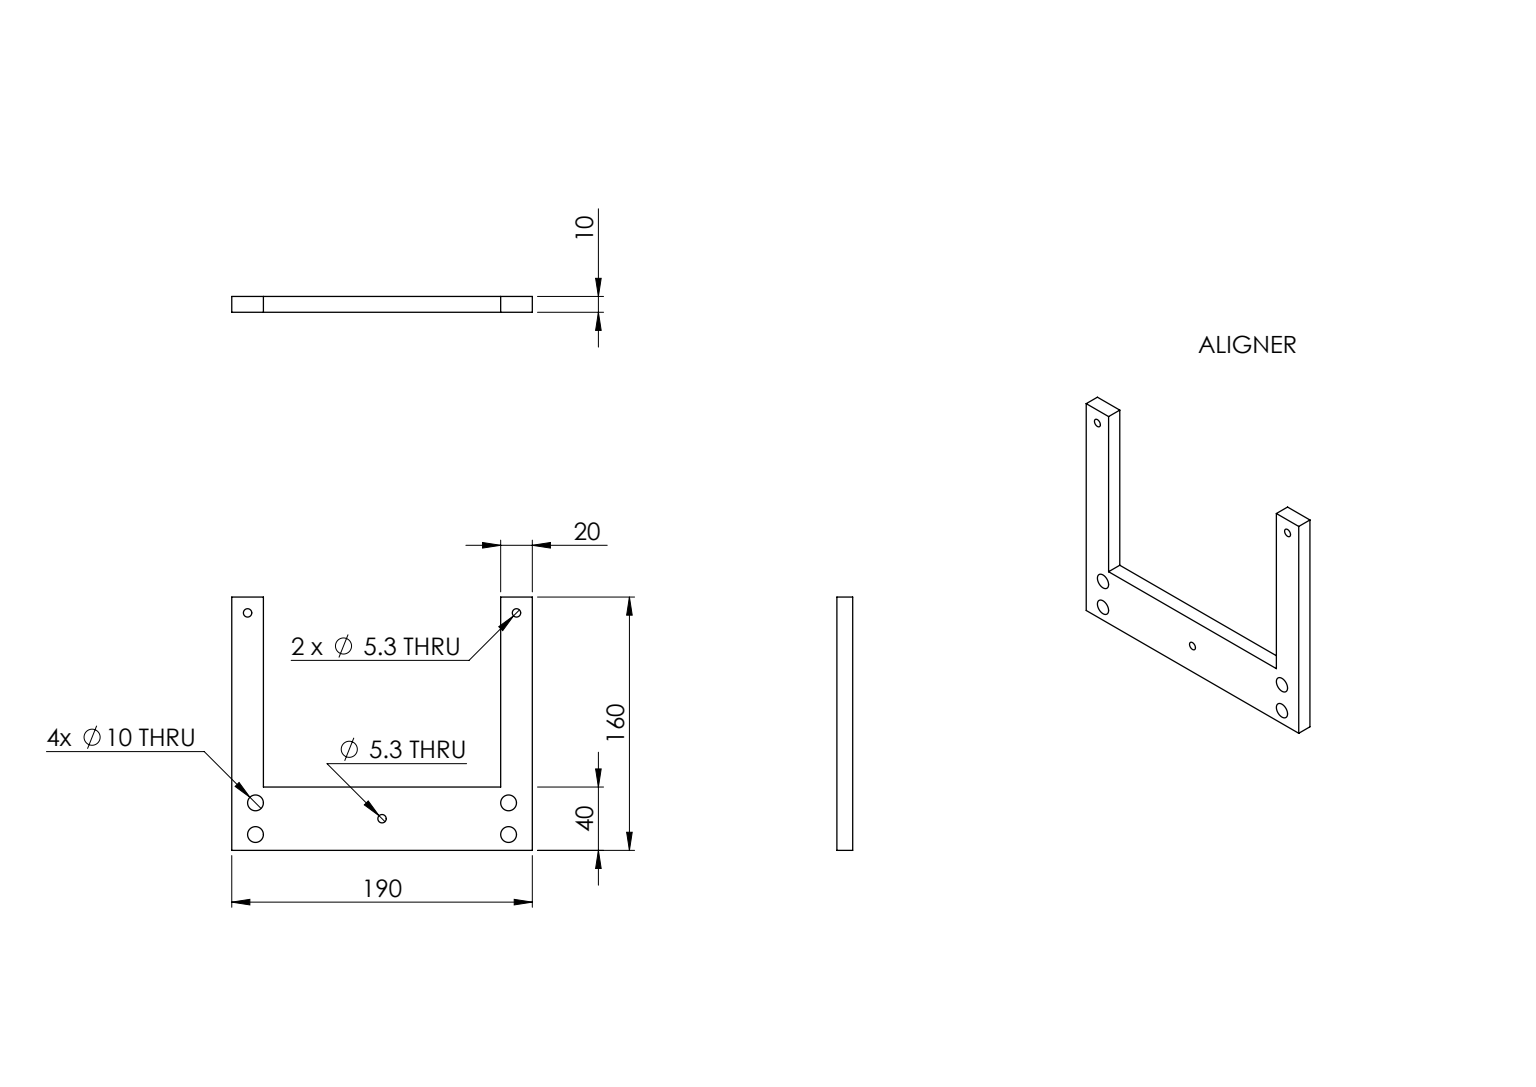
ISO-10303-21;
HEADER;
FILE_DESCRIPTION (('STEP AP214'),
    '1' );
FILE_NAME ('aligner.step',
    '2026-10-24T13:33:06',
    ( '' ),
    ( '' ),
    'SwSTEP 2.0',
    'SolidWorks 2026',
    '' );
FILE_SCHEMA (( 'AUTOMOTIVE_DESIGN' ));
ENDSEC;

DATA;
#23=ORIENTED_EDGE ( 'NONE', *, *, #5278, .F. ) ;
#39=ORIENTED_EDGE ( 'NONE', *, *, #7804, .T. ) ;
#91=ADVANCED_FACE ( 'NONE', ( #1003 ), #2259, .T. ) ;
#92=CARTESIAN_POINT ( 'NONE',  ( -144.9999999999999432, -105.0000000000000853, 40.00000000000000000 ) ) ;
#103=DIRECTION ( 'NONE',  ( -1.000000000000000000, 0.000000000000000000, 0.000000000000000000 ) ) ;
#109=SURFACE_STYLE_FILL_AREA ( #5656 ) ;
#110=EDGE_CURVE ( 'NONE', #13194, #10462, #10760, .T. ) ;
#136=EDGE_LOOP ( 'NONE', ( #496, #11440, #13448, #1824 ) ) ;
#153=PLANE ( 'NONE',  #6564 ) ;
#202=DIRECTION ( 'NONE',  ( -0.000000000000000000, 0.000000000000000000, -1.000000000000000000 ) ) ;
#219=CIRCLE ( 'NONE', #5381, 5.000000000000004441 ) ;
#220=AXIS2_PLACEMENT_3D ( 'NONE', #2707, #9091, #281 ) ;
#224=CARTESIAN_POINT ( 'NONE',  ( -219.9999999999999147, -85.00000000000009948, 30.00000000000000000 ) ) ;
#238=EDGE_CURVE ( 'NONE', #5881, #9436, #12617, .T. ) ;
#248=DIRECTION ( 'NONE',  ( -0.000000000000000000, -0.000000000000000000, -1.000000000000000000 ) ) ;
#250=DIRECTION ( 'NONE',  ( 1.000000000000000000, 0.000000000000000000, 0.000000000000000000 ) ) ;
#251=EDGE_CURVE ( 'NONE', #12108, #865, #13488, .T. ) ;
#281=DIRECTION ( 'NONE',  ( 0.000000000000000000, 0.000000000000000000, -1.000000000000000000 ) ) ;
#287=DIRECTION ( 'NONE',  ( -0.000000000000000000, -1.000000000000000000, -0.000000000000000000 ) ) ;
#291=PRODUCT_DEFINITION_SHAPE ( 'NONE', 'NONE',  #3819 ) ;
#312=CARTESIAN_POINT ( 'NONE',  ( -304.9999999999999432, 45.00000000000001421, 30.00000000000000000 ) ) ;
#323=EDGE_LOOP ( 'NONE', ( #13718, #1656 ) ) ;
#332=FACE_OUTER_BOUND ( 'NONE', #8846, .T. ) ;
#341=CIRCLE ( 'NONE', #14262, 2.649999999999985700 ) ;
#353=FACE_BOUND ( 'NONE', #877, .T. ) ;
#354=AXIS2_PLACEMENT_3D ( 'NONE', #6912, #4747, #11272 ) ;
#367=LINE ( 'NONE', #8152, #5578 ) ;
#369=MECHANICAL_DESIGN_GEOMETRIC_PRESENTATION_REPRESENTATION('',(#7806),#10136);
#403=ORIENTED_EDGE ( 'NONE', *, *, #10858, .T. ) ;
#413=ADVANCED_FACE ( 'NONE', ( #5943 ), #5008, .F. ) ;
#417=VERTEX_POINT ( 'NONE', #3915 ) ;
#420=ORIENTED_EDGE ( 'NONE', *, *, #110, .F. ) ;
#422=ORIENTED_EDGE ( 'NONE', *, *, #251, .T. ) ;
#432=AXIS2_PLACEMENT_3D ( 'NONE', #6019, #1877, #3778 ) ;
#438=ORIENTED_EDGE ( 'NONE', *, *, #6313, .F. ) ;
#442=DIRECTION ( 'NONE',  ( -1.000000000000000000, 0.000000000000000000, 0.000000000000000000 ) ) ;
#450=ADVANCED_FACE ( 'NONE', ( #1804 ), #8183, .F. ) ;
#473=AXIS2_PLACEMENT_3D ( 'NONE', #9647, #5162, #2982 ) ;
#475=DIRECTION ( 'NONE',  ( -1.000000000000000000, 0.000000000000000000, 0.000000000000000000 ) ) ;
#477=EDGE_LOOP ( 'NONE', ( #11769, #9508 ) ) ;
#479=CARTESIAN_POINT ( 'NONE',  ( -299.9999999999999432, -95.00000000000008527, 354.1421356237308942 ) ) ;
#496=ORIENTED_EDGE ( 'NONE', *, *, #11704, .F. ) ;
#499=DIRECTION ( 'NONE',  ( 0.000000000000000000, 0.000000000000000000, -1.000000000000000000 ) ) ;
#508=FACE_OUTER_BOUND ( 'NONE', #3187, .T. ) ;
#520=CARTESIAN_POINT ( 'NONE',  ( -144.9999999999999432, -105.0000000000000853, 40.00000000000000000 ) ) ;
#528=ADVANCED_FACE ( 'NONE', ( #2680 ), #11531, .F. ) ;
#543=LINE ( 'NONE', #10288, #10586 ) ;
#547=DIRECTION ( 'NONE',  ( 0.000000000000000000, -0.000000000000000000, 1.000000000000000000 ) ) ;
#555=ORIENTED_EDGE ( 'NONE', *, *, #6914, .F. ) ;
#575=DIRECTION ( 'NONE',  ( 1.000000000000000000, 7.304098846218135653E-17, -0.000000000000000000 ) ) ;
#592=PLANE ( 'NONE',  #11528 ) ;
#598=AXIS2_PLACEMENT_3D ( 'NONE', #11123, #1157, #11993 ) ;
#606=ORIENTED_EDGE ( 'NONE', *, *, #1377, .T. ) ;
#608=AXIS2_PLACEMENT_3D ( 'NONE', #4664, #202, #3506 ) ;
#609=LINE ( 'NONE', #2598, #1621 ) ;
#652=ORIENTED_EDGE ( 'NONE', *, *, #7099, .T. ) ;
#663=VERTEX_POINT ( 'NONE', #2017 ) ;
#740=CARTESIAN_POINT ( 'NONE',  ( -304.9999999999999432, -75.00000000000008527, 39.99999999999997868 ) ) ;
#741=CYLINDRICAL_SURFACE ( 'NONE', #5392, 2.649999999999985700 ) ;
#775=DIRECTION ( 'NONE',  ( -1.000000000000000000, 0.000000000000000000, 0.000000000000000000 ) ) ;
#777=ORIENTED_EDGE ( 'NONE', *, *, #7329, .T. ) ;
#820=EDGE_LOOP ( 'NONE', ( #4312, #1747, #10761, #1441 ) ) ;
#852=( LENGTH_UNIT ( ) NAMED_UNIT ( * ) SI_UNIT ( .MILLI., .METRE. ) );
#863=EDGE_LOOP ( 'NONE', ( #12473, #1825 ) ) ;
#865=VERTEX_POINT ( 'NONE', #13683 ) ;
#877=EDGE_LOOP ( 'NONE', ( #5483, #13862 ) ) ;
#904=ORIENTED_EDGE ( 'NONE', *, *, #1524, .T. ) ;
#971=AXIS2_PLACEMENT_3D ( 'NONE', #12444, #13808, #8300 ) ;
#981=VERTEX_POINT ( 'NONE', #9708 ) ;
#998=DIRECTION ( 'NONE',  ( 1.000000000000000000, 0.000000000000000000, 0.000000000000000000 ) ) ;
#1003=FACE_OUTER_BOUND ( 'NONE', #2000, .T. ) ;
#1034=CIRCLE ( 'NONE', #14250, 5.000000000000004441 ) ;
#1087=DIRECTION ( 'NONE',  ( 0.000000000000000000, 1.000000000000000000, 0.000000000000000000 ) ) ;
#1090=CARTESIAN_POINT ( 'NONE',  ( -140.0000000000000000, -95.00000000000008527, 40.00000000000000000 ) ) ;
#1122=VECTOR ( 'NONE', #11092, 1000.000000000000000 ) ;
#1157=DIRECTION ( 'NONE',  ( -0.000000000000000000, -0.000000000000000000, -1.000000000000000000 ) ) ;
#1160=CYLINDRICAL_SURFACE ( 'NONE', #8697, 5.000000000000004441 ) ;
#1167=CARTESIAN_POINT ( 'NONE',  ( -314.9999999999999432, 55.00000000000001421, 30.00000000000000000 ) ) ;
#1174=ADVANCED_FACE ( 'NONE', ( #7983 ), #4410, .T. ) ;
#1191=VECTOR ( 'NONE', #7717, 1000.000000000000000 ) ;
#1214=DIRECTION ( 'NONE',  ( 0.000000000000000000, -0.000000000000000000, 1.000000000000000000 ) ) ;
#1247=CARTESIAN_POINT ( 'NONE',  ( -124.9999999999999432, -105.0000000000000853, 40.00000000000000000 ) ) ;
#1276=ORIENTED_EDGE ( 'NONE', *, *, #9037, .T. ) ;
#1299=EDGE_CURVE ( 'NONE', #13972, #8006, #4015, .T. ) ;
#1300=CIRCLE ( 'NONE', #6183, 5.000000000000004441 ) ;
#1347=PRODUCT ( 'aligner', 'aligner', '', ( #6175 ) ) ;
#1353=CARTESIAN_POINT ( 'NONE',  ( -314.9999999999999432, -105.0000000000000995, 40.00000000000000000 ) ) ;
#1354=DIRECTION ( 'NONE',  ( -0.000000000000000000, -0.000000000000000000, -1.000000000000000000 ) ) ;
#1377=EDGE_CURVE ( 'NONE', #5028, #10577, #8861, .T. ) ;
#1406=CARTESIAN_POINT ( 'NONE',  ( -294.9999999999999432, -75.00000000000008527, 39.99999999999997868 ) ) ;
#1414=DIRECTION ( 'NONE',  ( -0.000000000000000000, -0.000000000000000000, -1.000000000000000000 ) ) ;
#1441=ORIENTED_EDGE ( 'NONE', *, *, #12534, .T. ) ;
#1459=ORIENTED_EDGE ( 'NONE', *, *, #6313, .T. ) ;
#1512=EDGE_CURVE ( 'NONE', #4493, #865, #13215, .T. ) ;
#1524=EDGE_CURVE ( 'NONE', #6598, #3716, #12128, .T. ) ;
#1530=AXIS2_PLACEMENT_3D ( 'NONE', #9386, #12937, #7060 ) ;
#1569=CARTESIAN_POINT ( 'NONE',  ( -140.0000000000000000, -75.00000000000008527, 30.00000000000000000 ) ) ;
#1582=ORIENTED_EDGE ( 'NONE', *, *, #8645, .T. ) ;
#1621=VECTOR ( 'NONE', #6943, 1000.000000000000000 ) ;
#1631=CARTESIAN_POINT ( 'NONE',  ( -134.9999999999999716, 45.00000000000001421, 30.00000000000000000 ) ) ;
#1649=CIRCLE ( 'NONE', #473, 5.000000000000004441 ) ;
#1653=ORIENTED_EDGE ( 'NONE', *, *, #8448, .T. ) ;
#1655=CYLINDRICAL_SURFACE ( 'NONE', #5562, 5.000000000000004441 ) ;
#1656=ORIENTED_EDGE ( 'NONE', *, *, #12195, .T. ) ;
#1691=CARTESIAN_POINT ( 'NONE',  ( -294.9999999999999432, -75.00000000000008527, 354.1421356237308942 ) ) ;
#1695=EDGE_CURVE ( 'NONE', #7212, #9436, #2619, .T. ) ;
#1718=DIRECTION ( 'NONE',  ( -0.000000000000000000, 0.000000000000000000, -1.000000000000000000 ) ) ;
#1723=CARTESIAN_POINT ( 'NONE',  ( -299.9999999999999432, -75.00000000000008527, 354.1421356237308942 ) ) ;
#1725=DIRECTION ( 'NONE',  ( -0.000000000000000000, -0.000000000000000000, -1.000000000000000000 ) ) ;
#1745=ORIENTED_EDGE ( 'NONE', *, *, #4492, .F. ) ;
#1747=ORIENTED_EDGE ( 'NONE', *, *, #5401, .T. ) ;
#1766=CARTESIAN_POINT ( 'NONE',  ( -294.9999999999999432, -65.00000000000011369, 30.00000000000000000 ) ) ;
#1773=FACE_BOUND ( 'NONE', #3437, .T. ) ;
#1781=ORIENTED_EDGE ( 'NONE', *, *, #1695, .T. ) ;
#1804=FACE_OUTER_BOUND ( 'NONE', #8996, .T. ) ;
#1810=VERTEX_POINT ( 'NONE', #2905 ) ;
#1824=ORIENTED_EDGE ( 'NONE', *, *, #4456, .T. ) ;
#1825=ORIENTED_EDGE ( 'NONE', *, *, #5920, .F. ) ;
#1875=ORIENTED_EDGE ( 'NONE', *, *, #7549, .T. ) ;
#1877=DIRECTION ( 'NONE',  ( -0.000000000000000000, 0.000000000000000000, -1.000000000000000000 ) ) ;
#1878=EDGE_CURVE ( 'NONE', #13081, #11113, #4181, .T. ) ;
#1879=ADVANCED_FACE ( 'NONE', ( #10446 ), #1655, .F. ) ;
#1887=CARTESIAN_POINT ( 'NONE',  ( -219.9999999999999147, -85.00000000000009948, 30.00000000000000000 ) ) ;
#1965=CARTESIAN_POINT ( 'NONE',  ( -124.9999999999999432, 55.00000000000001421, 40.00000000000000000 ) ) ;
#1973=DIRECTION ( 'NONE',  ( -1.000000000000000000, -7.304098846218135653E-17, 0.000000000000000000 ) ) ;
#1975=DIRECTION ( 'NONE',  ( -0.000000000000000000, 0.000000000000000000, -1.000000000000000000 ) ) ;
#1978=AXIS2_PLACEMENT_3D ( 'NONE', #6016, #10442, #475 ) ;
#1982=VERTEX_POINT ( 'NONE', #12040 ) ;
#1987=FACE_OUTER_BOUND ( 'NONE', #13855, .T. ) ;
#1993=FACE_BOUND ( 'NONE', #863, .T. ) ;
#2000=EDGE_LOOP ( 'NONE', ( #1745, #12037, #3225, #9323 ) ) ;
#2004=VECTOR ( 'NONE', #287, 1000.000000000000000 ) ;
#2017=CARTESIAN_POINT ( 'NONE',  ( -307.6499999999999204, 45.00000000000001421, 40.00000000000000000 ) ) ;
#2064=CARTESIAN_POINT ( 'NONE',  ( -294.9999999999999432, -65.00000000000011369, 40.00000000000000000 ) ) ;
#2072=DIRECTION ( 'NONE',  ( -1.000000000000000000, 0.000000000000000000, 0.000000000000000000 ) ) ;
#2098=EDGE_LOOP ( 'NONE', ( #8207, #7792 ) ) ;
#2112=ORIENTED_EDGE ( 'NONE', *, *, #1524, .F. ) ;
#2125=CIRCLE ( 'NONE', #3735, 2.649999999999985700 ) ;
#2137=ORIENTED_EDGE ( 'NONE', *, *, #7283, .T. ) ;
#2148=LINE ( 'NONE', #2289, #6717 ) ;
#2186=DIRECTION ( 'NONE',  ( -1.000000000000000000, -1.460819769243627131E-16, 0.000000000000000000 ) ) ;
#2211=DIRECTION ( 'NONE',  ( -1.000000000000000000, 0.000000000000000000, 0.000000000000000000 ) ) ;
#2239=VERTEX_POINT ( 'NONE', #7655 ) ;
#2248=AXIS2_PLACEMENT_3D ( 'NONE', #13499, #6762, #4521 ) ;
#2259=PLANE ( 'NONE',  #4981 ) ;
#2262=CIRCLE ( 'NONE', #7126, 2.649999999999985700 ) ;
#2265=ORIENTED_EDGE ( 'NONE', *, *, #5401, .F. ) ;
#2271=DIRECTION ( 'NONE',  ( -0.000000000000000000, 0.000000000000000000, -1.000000000000000000 ) ) ;
#2289=CARTESIAN_POINT ( 'NONE',  ( -132.3499999999999943, 45.00000000000001421, 30.00000000000000000 ) ) ;
#2322=FILL_AREA_STYLE_COLOUR ( '', #10495 ) ;
#2336=VERTEX_POINT ( 'NONE', #4687 ) ;
#2355=DIRECTION ( 'NONE',  ( 1.000000000000000000, 0.000000000000000000, 0.000000000000000000 ) ) ;
#2382=PRODUCT_DEFINITION_FORMATION_WITH_SPECIFIED_SOURCE ( 'ANY', '', #1347, .NOT_KNOWN. ) ;
#2383=ORIENTED_EDGE ( 'NONE', *, *, #12018, .T. ) ;
#2389=VECTOR ( 'NONE', #11604, 1000.000000000000000 ) ;
#2401=ORIENTED_EDGE ( 'NONE', *, *, #6755, .F. ) ;
#2408=CARTESIAN_POINT ( 'NONE',  ( -144.9999999999999432, -105.0000000000000853, 30.00000000000000000 ) ) ;
#2415=ORIENTED_EDGE ( 'NONE', *, *, #10083, .F. ) ;
#2468=ORIENTED_EDGE ( 'NONE', *, *, #13310, .F. ) ;
#2505=LINE ( 'NONE', #6918, #8854 ) ;
#2507=LINE ( 'NONE', #3524, #6486 ) ;
#2513=EDGE_CURVE ( 'NONE', #13072, #981, #4528, .T. ) ;
#2533=VECTOR ( 'NONE', #11742, 1000.000000000000000 ) ;
#2540=VERTEX_POINT ( 'NONE', #12002 ) ;
#2577=DIRECTION ( 'NONE',  ( -0.000000000000000000, -0.000000000000000000, -1.000000000000000000 ) ) ;
#2598=CARTESIAN_POINT ( 'NONE',  ( -124.9999999999999432, -65.00000000000008527, 30.00000000000000000 ) ) ;
#2609=DIRECTION ( 'NONE',  ( 1.000000000000000000, 0.000000000000000000, 0.000000000000000000 ) ) ;
#2613=EDGE_LOOP ( 'NONE', ( #438, #8269, #2615, #12189 ) ) ;
#2615=ORIENTED_EDGE ( 'NONE', *, *, #10294, .T. ) ;
#2619=LINE ( 'NONE', #10158, #7237 ) ;
#2679=ORIENTED_EDGE ( 'NONE', *, *, #12960, .F. ) ;
#2680=FACE_OUTER_BOUND ( 'NONE', #6752, .T. ) ;
#2707=CARTESIAN_POINT ( 'NONE',  ( -294.9999999999999432, -105.0000000000000853, 40.00000000000000000 ) ) ;
#2779=ORIENTED_EDGE ( 'NONE', *, *, #6667, .T. ) ;
#2787=PLANE ( 'NONE',  #9424 ) ;
#2801=ORIENTED_EDGE ( 'NONE', *, *, #4387, .T. ) ;
#2833=VECTOR ( 'NONE', #3291, 1000.000000000000000 ) ;
#2853=ORIENTED_EDGE ( 'NONE', *, *, #2513, .F. ) ;
#2887=VERTEX_POINT ( 'NONE', #5103 ) ;
#2895=LINE ( 'NONE', #9572, #2533 ) ;
#2905=CARTESIAN_POINT ( 'NONE',  ( -222.6499999999998920, -85.00000000000009948, 30.00000000000000000 ) ) ;
#2909=EDGE_LOOP ( 'NONE', ( #12132, #1459, #6840, #3447 ) ) ;
#2927=FACE_OUTER_BOUND ( 'NONE', #11134, .T. ) ;
#2930=FACE_BOUND ( 'NONE', #10179, .T. ) ;
#2942=CIRCLE ( 'NONE', #3179, 5.000000000000004441 ) ;
#2949=CARTESIAN_POINT ( 'NONE',  ( -144.9999999999999432, -65.00000000000008527, 40.00000000000000000 ) ) ;
#2982=DIRECTION ( 'NONE',  ( 1.000000000000000000, 0.000000000000000000, 0.000000000000000000 ) ) ;
#3019=ORIENTED_EDGE ( 'NONE', *, *, #1299, .T. ) ;
#3021=CARTESIAN_POINT ( 'NONE',  ( -314.9999999999999432, -105.0000000000000995, 40.00000000000000000 ) ) ;
#3028=FACE_BOUND ( 'NONE', #9601, .T. ) ;
#3040=ORIENTED_EDGE ( 'NONE', *, *, #11028, .F. ) ;
#3062=CARTESIAN_POINT ( 'NONE',  ( -132.3499999999999943, 45.00000000000001421, 30.00000000000000000 ) ) ;
#3106=FACE_BOUND ( 'NONE', #12537, .T. ) ;
#3120=DIRECTION ( 'NONE',  ( 1.000000000000000000, 0.000000000000000000, 0.000000000000000000 ) ) ;
#3123=ORIENTED_EDGE ( 'NONE', *, *, #6292, .T. ) ;
#3179=AXIS2_PLACEMENT_3D ( 'NONE', #8521, #6352, #10782 ) ;
#3187=EDGE_LOOP ( 'NONE', ( #1582, #6980, #3939, #6808 ) ) ;
#3211=VECTOR ( 'NONE', #9099, 1000.000000000000000 ) ;
#3225=ORIENTED_EDGE ( 'NONE', *, *, #10052, .T. ) ;
#3246=VECTOR ( 'NONE', #13387, 1000.000000000000000 ) ;
#3291=DIRECTION ( 'NONE',  ( 1.000000000000000000, 7.304098846218135653E-17, -0.000000000000000000 ) ) ;
#3321=CARTESIAN_POINT ( 'NONE',  ( -304.9999999999999432, 45.00000000000001421, 30.00000000000000000 ) ) ;
#3339=EDGE_CURVE ( 'NONE', #2239, #5230, #5127, .T. ) ;
#3369=DIRECTION ( 'NONE',  ( -0.000000000000000000, 0.000000000000000000, -1.000000000000000000 ) ) ;
#3373=DIRECTION ( 'NONE',  ( 1.000000000000000000, 0.000000000000000000, 0.000000000000000000 ) ) ;
#3437=EDGE_LOOP ( 'NONE', ( #13630, #12058 ) ) ;
#3447=ORIENTED_EDGE ( 'NONE', *, *, #10294, .F. ) ;
#3457=CIRCLE ( 'NONE', #6920, 5.000000000000004441 ) ;
#3464=DIRECTION ( 'NONE',  ( 0.000000000000000000, 1.000000000000000000, 0.000000000000000000 ) ) ;
#3506=DIRECTION ( 'NONE',  ( 1.000000000000000000, 0.000000000000000000, 0.000000000000000000 ) ) ;
#3524=CARTESIAN_POINT ( 'NONE',  ( -307.6499999999999204, 45.00000000000001421, 30.00000000000000000 ) ) ;
#3560=CARTESIAN_POINT ( 'NONE',  ( -124.9999999999999432, -105.0000000000000853, 40.00000000000000000 ) ) ;
#3627=CIRCLE ( 'NONE', #8729, 5.000000000000004441 ) ;
#3639=CIRCLE ( 'NONE', #598, 2.649999999999985700 ) ;
#3708=DIRECTION ( 'NONE',  ( -0.000000000000000000, -0.000000000000000000, -1.000000000000000000 ) ) ;
#3716=VERTEX_POINT ( 'NONE', #1167 ) ;
#3724=FACE_BOUND ( 'NONE', #323, .T. ) ;
#3727=LINE ( 'NONE', #9923, #2004 ) ;
#3731=CARTESIAN_POINT ( 'NONE',  ( -307.6499999999999204, 45.00000000000001421, 30.00000000000000000 ) ) ;
#3735=AXIS2_PLACEMENT_3D ( 'NONE', #5207, #9622, #2072 ) ;
#3764=CARTESIAN_POINT ( 'NONE',  ( -124.9999999999999432, 55.00000000000001421, 30.00000000000000000 ) ) ;
#3778=DIRECTION ( 'NONE',  ( 1.000000000000000000, 0.000000000000000000, 0.000000000000000000 ) ) ;
#3799=LINE ( 'NONE', #9315, #10831 ) ;
#3809=DIRECTION ( 'NONE',  ( -0.000000000000000000, -0.000000000000000000, -1.000000000000000000 ) ) ;
#3810=CLOSED_SHELL ( 'NONE', ( #7980, #528, #10284, #12528, #450, #11788, #1879, #11864, #12453, #9342, #5261, #6691, #9234, #1174, #4628, #13130, #91, #6937, #10572, #13117, #413, #6012, #13880, #14110 ) ) ;
#3818=CYLINDRICAL_SURFACE ( 'NONE', #10112, 2.649999999999985700 ) ;
#3819=PRODUCT_DEFINITION ( 'UNKNOWN', '', #2382, #6290 ) ;
#3864=CIRCLE ( 'NONE', #11976, 2.649999999999985700 ) ;
#3877=LINE ( 'NONE', #4090, #7803 ) ;
#3915=CARTESIAN_POINT ( 'NONE',  ( -217.3499999999999375, -85.00000000000009948, 30.00000000000000000 ) ) ;
#3939=ORIENTED_EDGE ( 'NONE', *, *, #5202, .T. ) ;
#3953=DIRECTION ( 'NONE',  ( -0.000000000000000000, -0.000000000000000000, -1.000000000000000000 ) ) ;
#3963=FACE_BOUND ( 'NONE', #14205, .T. ) ;
#3986=EDGE_CURVE ( 'NONE', #6598, #13972, #13276, .T. ) ;
#4015=LINE ( 'NONE', #7129, #10195 ) ;
#4057=DIRECTION ( 'NONE',  ( 1.000000000000000000, 0.000000000000000000, 0.000000000000000000 ) ) ;
#4065=DIRECTION ( 'NONE',  ( 0.000000000000000000, -0.000000000000000000, 1.000000000000000000 ) ) ;
#4085=AXIS2_PLACEMENT_3D ( 'NONE', #6459, #4065, #11759 ) ;
#4090=CARTESIAN_POINT ( 'NONE',  ( -217.3499999999999375, -85.00000000000009948, 30.00000000000000000 ) ) ;
#4102=DIRECTION ( 'NONE',  ( -0.000000000000000000, -0.000000000000000000, -1.000000000000000000 ) ) ;
#4124=ORIENTED_EDGE ( 'NONE', *, *, #3339, .F. ) ;
#4136=DIRECTION ( 'NONE',  ( -0.000000000000000000, 0.000000000000000000, -1.000000000000000000 ) ) ;
#4181=CIRCLE ( 'NONE', #432, 5.000000000000004441 ) ;
#4188=VECTOR ( 'NONE', #12173, 1000.000000000000000 ) ;
#4218=LINE ( 'NONE', #12050, #11760 ) ;
#4228=DIRECTION ( 'NONE',  ( 0.000000000000000000, -0.000000000000000000, 1.000000000000000000 ) ) ;
#4256=VERTEX_POINT ( 'NONE', #8178 ) ;
#4257=FACE_BOUND ( 'NONE', #9141, .T. ) ;
#4290=DIRECTION ( 'NONE',  ( 0.000000000000000000, 0.000000000000000000, -1.000000000000000000 ) ) ;
#4295=CARTESIAN_POINT ( 'NONE',  ( -140.0000000000000000, -75.00000000000008527, 40.00000000000000000 ) ) ;
#4312=ORIENTED_EDGE ( 'NONE', *, *, #5068, .F. ) ;
#4343=CIRCLE ( 'NONE', #10844, 2.649999999999985700 ) ;
#4359=UNCERTAINTY_MEASURE_WITH_UNIT (LENGTH_MEASURE( 1.000000000000000082E-05 ), #7754, 'distance_accuracy_value', 'NONE');
#4379=DIRECTION ( 'NONE',  ( -1.000000000000000000, 0.000000000000000000, 0.000000000000000000 ) ) ;
#4387=EDGE_CURVE ( 'NONE', #7915, #7212, #3457, .T. ) ;
#4410=PLANE ( 'NONE',  #220 ) ;
#4437=( NAMED_UNIT ( * ) SI_UNIT ( $, .STERADIAN. ) SOLID_ANGLE_UNIT ( ) );
#4451=LINE ( 'NONE', #2408, #11517 ) ;
#4456=EDGE_CURVE ( 'NONE', #13972, #10462, #2895, .T. ) ;
#4459=ORIENTED_EDGE ( 'NONE', *, *, #10381, .T. ) ;
#4479=( GEOMETRIC_REPRESENTATION_CONTEXT ( 3 ) GLOBAL_UNCERTAINTY_ASSIGNED_CONTEXT ( ( #9868 ) ) GLOBAL_UNIT_ASSIGNED_CONTEXT ( ( #5519, #4648, #4437 ) ) REPRESENTATION_CONTEXT ( 'NONE', 'WORKASPACE' ) );
#4492=EDGE_CURVE ( 'NONE', #12063, #9564, #13320, .T. ) ;
#4493=VERTEX_POINT ( 'NONE', #7801 ) ;
#4521=DIRECTION ( 'NONE',  ( 1.000000000000000000, 0.000000000000000000, 0.000000000000000000 ) ) ;
#4528=CIRCLE ( 'NONE', #12618, 5.000000000000004441 ) ;
#4535=EDGE_CURVE ( 'NONE', #11936, #11113, #8762, .T. ) ;
#4586=FACE_OUTER_BOUND ( 'NONE', #14222, .T. ) ;
#4606=DIRECTION ( 'NONE',  ( 0.000000000000000000, 0.000000000000000000, 1.000000000000000000 ) ) ;
#4620=LINE ( 'NONE', #10197, #8516 ) ;
#4623=PLANE ( 'NONE',  #6927 ) ;
#4628=ADVANCED_FACE ( 'NONE', ( #8088 ), #4623, .T. ) ;
#4648=( NAMED_UNIT ( * ) PLANE_ANGLE_UNIT ( ) SI_UNIT ( $, .RADIAN. ) );
#4664=CARTESIAN_POINT ( 'NONE',  ( -140.0000000000000000, -95.00000000000008527, 30.00000000000000000 ) ) ;
#4675=LINE ( 'NONE', #8331, #2389 ) ;
#4687=CARTESIAN_POINT ( 'NONE',  ( -132.3499999999999943, 45.00000000000001421, 40.00000000000000000 ) ) ;
#4695=VECTOR ( 'NONE', #3809, 1000.000000000000000 ) ;
#4747=DIRECTION ( 'NONE',  ( -0.000000000000000000, 0.000000000000000000, -1.000000000000000000 ) ) ;
#4763=EDGE_LOOP ( 'NONE', ( #1653, #5160, #10543, #904 ) ) ;
#4775=CIRCLE ( 'NONE', #4085, 2.649999999999985700 ) ;
#4802=CARTESIAN_POINT ( 'NONE',  ( -304.9999999999999432, 45.00000000000001421, 30.00000000000000000 ) ) ;
#4824=FACE_OUTER_BOUND ( 'NONE', #8526, .T. ) ;
#4861=DIRECTION ( 'NONE',  ( -0.000000000000000000, -0.000000000000000000, -1.000000000000000000 ) ) ;
#4873=EDGE_LOOP ( 'NONE', ( #23, #555, #6683, #2383 ) ) ;
#4902=DIRECTION ( 'NONE',  ( -0.000000000000000000, -0.000000000000000000, -1.000000000000000000 ) ) ;
#4912=VERTEX_POINT ( 'NONE', #6713 ) ;
#4917=DIRECTION ( 'NONE',  ( 0.000000000000000000, -0.000000000000000000, 1.000000000000000000 ) ) ;
#4943=DIRECTION ( 'NONE',  ( -0.000000000000000000, -0.000000000000000000, -1.000000000000000000 ) ) ;
#4965=ORIENTED_EDGE ( 'NONE', *, *, #1512, .T. ) ;
#4966=FACE_BOUND ( 'NONE', #2098, .T. ) ;
#4979=FACE_OUTER_BOUND ( 'NONE', #9904, .T. ) ;
#4981=AXIS2_PLACEMENT_3D ( 'NONE', #1965, #8863, #4228 ) ;
#4982=DIRECTION ( 'NONE',  ( -1.000000000000000000, 0.000000000000000000, 0.000000000000000000 ) ) ;
#5008=CYLINDRICAL_SURFACE ( 'NONE', #13087, 5.000000000000004441 ) ;
#5028=VERTEX_POINT ( 'NONE', #8674 ) ;
#5061=FACE_OUTER_BOUND ( 'NONE', #8591, .T. ) ;
#5068=EDGE_CURVE ( 'NONE', #2336, #14079, #2148, .T. ) ;
#5075=ORIENTED_EDGE ( 'NONE', *, *, #11318, .T. ) ;
#5077=DIRECTION ( 'NONE',  ( 1.000000000000000000, 0.000000000000000000, 0.000000000000000000 ) ) ;
#5081=EDGE_CURVE ( 'NONE', #663, #5230, #2507, .T. ) ;
#5087=DIRECTION ( 'NONE',  ( -0.000000000000000000, -0.000000000000000000, -1.000000000000000000 ) ) ;
#5103=CARTESIAN_POINT ( 'NONE',  ( -304.9999999999999432, -95.00000000000008527, 39.99999999999997868 ) ) ;
#5124=DIRECTION ( 'NONE',  ( 1.460819769243627131E-16, -1.000000000000000000, 0.000000000000000000 ) ) ;
#5125=ORIENTED_EDGE ( 'NONE', *, *, #7329, .F. ) ;
#5127=CIRCLE ( 'NONE', #13220, 2.649999999999985700 ) ;
#5158=DIRECTION ( 'NONE',  ( -1.000000000000000000, 0.000000000000000000, 0.000000000000000000 ) ) ;
#5160=ORIENTED_EDGE ( 'NONE', *, *, #7549, .F. ) ;
#5162=DIRECTION ( 'NONE',  ( -0.000000000000000000, 0.000000000000000000, -1.000000000000000000 ) ) ;
#5202=EDGE_CURVE ( 'NONE', #417, #1810, #13195, .T. ) ;
#5207=CARTESIAN_POINT ( 'NONE',  ( -134.9999999999999716, 45.00000000000001421, 30.00000000000000000 ) ) ;
#5215=CARTESIAN_POINT ( 'NONE',  ( -144.9999999999999432, -65.00000000000008527, 30.00000000000000000 ) ) ;
#5218=CARTESIAN_POINT ( 'NONE',  ( -137.6499999999999773, 45.00000000000001421, 40.00000000000000000 ) ) ;
#5228=CARTESIAN_POINT ( 'NONE',  ( -314.9999999999999432, 55.00000000000001421, 30.00000000000000000 ) ) ;
#5230=VERTEX_POINT ( 'NONE', #3731 ) ;
#5241=CARTESIAN_POINT ( 'NONE',  ( -145.0000000000000284, -75.00000000000008527, 40.00000000000000000 ) ) ;
#5242=VECTOR ( 'NONE', #3708, 1000.000000000000000 ) ;
#5259=AXIS2_PLACEMENT_3D ( 'NONE', #1887, #10749, #775 ) ;
#5261=ADVANCED_FACE ( 'NONE', ( #10117 ), #153, .F. ) ;
#5278=EDGE_CURVE ( 'NONE', #13138, #13081, #11710, .T. ) ;
#5366=EDGE_CURVE ( 'NONE', #5028, #417, #3877, .T. ) ;
#5370=LINE ( 'NONE', #5228, #12789 ) ;
#5381=AXIS2_PLACEMENT_3D ( 'NONE', #10741, #4136, #13190 ) ;
#5392=AXIS2_PLACEMENT_3D ( 'NONE', #14026, #4102, #442 ) ;
#5401=EDGE_CURVE ( 'NONE', #2336, #7714, #4343, .T. ) ;
#5462=CIRCLE ( 'NONE', #14022, 5.000000000000004441 ) ;
#5471=DIRECTION ( 'NONE',  ( -0.000000000000000000, 0.000000000000000000, -1.000000000000000000 ) ) ;
#5480=DIRECTION ( 'NONE',  ( -0.000000000000000000, -0.000000000000000000, -1.000000000000000000 ) ) ;
#5483=ORIENTED_EDGE ( 'NONE', *, *, #2513, .T. ) ;
#5509=CARTESIAN_POINT ( 'NONE',  ( -219.9999999999999147, -85.00000000000009948, 30.00000000000000000 ) ) ;
#5519=( LENGTH_UNIT ( ) NAMED_UNIT ( * ) SI_UNIT ( .MILLI., .METRE. ) );
#5523=ORIENTED_EDGE ( 'NONE', *, *, #8204, .T. ) ;
#5528=ORIENTED_EDGE ( 'NONE', *, *, #5366, .F. ) ;
#5532=ORIENTED_EDGE ( 'NONE', *, *, #6667, .F. ) ;
#5534=ORIENTED_EDGE ( 'NONE', *, *, #1695, .F. ) ;
#5562=AXIS2_PLACEMENT_3D ( 'NONE', #479, #4943, #6094 ) ;
#5563=CARTESIAN_POINT ( 'NONE',  ( -294.9999999999999432, -75.00000000000008527, 30.00000000000002842 ) ) ;
#5578=VECTOR ( 'NONE', #9252, 1000.000000000000000 ) ;
#5609=DIRECTION ( 'NONE',  ( 1.000000000000000000, 0.000000000000000000, 0.000000000000000000 ) ) ;
#5656=FILL_AREA_STYLE ('',( #2322 ) ) ;
#5667=DIRECTION ( 'NONE',  ( 1.000000000000000000, 0.000000000000000000, 0.000000000000000000 ) ) ;
#5678=ORIENTED_EDGE ( 'NONE', *, *, #4535, .F. ) ;
#5697=LINE ( 'NONE', #13381, #7231 ) ;
#5700=VECTOR ( 'NONE', #9272, 1000.000000000000000 ) ;
#5705=AXIS2_PLACEMENT_3D ( 'NONE', #12057, #7483, #10757 ) ;
#5727=AXIS2_PLACEMENT_3D ( 'NONE', #4802, #8121, #5813 ) ;
#5740=CARTESIAN_POINT ( 'NONE',  ( -294.9999999999999432, 55.00000000000001421, 40.00000000000000000 ) ) ;
#5758=DIRECTION ( 'NONE',  ( -0.000000000000000000, -0.000000000000000000, -1.000000000000000000 ) ) ;
#5771=DIRECTION ( 'NONE',  ( 0.000000000000000000, -0.000000000000000000, 1.000000000000000000 ) ) ;
#5813=DIRECTION ( 'NONE',  ( -1.000000000000000000, 0.000000000000000000, 0.000000000000000000 ) ) ;
#5843=LINE ( 'NONE', #7936, #13260 ) ;
#5881=VERTEX_POINT ( 'NONE', #5241 ) ;
#5890=SHAPE_DEFINITION_REPRESENTATION ( #291, #9778 ) ;
#5920=EDGE_CURVE ( 'NONE', #4912, #2540, #9656, .T. ) ;
#5925=EDGE_CURVE ( 'NONE', #13138, #11936, #9176, .T. ) ;
#5943=FACE_OUTER_BOUND ( 'NONE', #4873, .T. ) ;
#5979=CARTESIAN_POINT ( 'NONE',  ( -145.0000000000000284, -75.00000000000008527, 30.00000000000000000 ) ) ;
#5992=ORIENTED_EDGE ( 'NONE', *, *, #11550, .T. ) ;
#6012=ADVANCED_FACE ( 'NONE', ( #8164 ), #3818, .F. ) ;
#6016=CARTESIAN_POINT ( 'NONE',  ( -304.9999999999999432, 45.00000000000001421, 30.00000000000000000 ) ) ;
#6019=CARTESIAN_POINT ( 'NONE',  ( -299.9999999999999432, -75.00000000000008527, 30.00000000000002842 ) ) ;
#6057=AXIS2_PLACEMENT_3D ( 'NONE', #7927, #12366, #4606 ) ;
#6062=DIRECTION ( 'NONE',  ( 0.000000000000000000, -0.000000000000000000, 1.000000000000000000 ) ) ;
#6088=MECHANICAL_DESIGN_GEOMETRIC_PRESENTATION_REPRESENTATION('',(#12571),#7448);
#6094=DIRECTION ( 'NONE',  ( -1.000000000000000000, 0.000000000000000000, 0.000000000000000000 ) ) ;
#6167=LINE ( 'NONE', #12622, #5242 ) ;
#6175=PRODUCT_CONTEXT ( 'NONE', #10266, 'mechanical' ) ;
#6183=AXIS2_PLACEMENT_3D ( 'NONE', #6799, #9113, #11224 ) ;
#6205=DIRECTION ( 'NONE',  ( 1.000000000000000000, 0.000000000000000000, 0.000000000000000000 ) ) ;
#6256=CARTESIAN_POINT ( 'NONE',  ( -219.9999999999999147, -85.00000000000009948, 40.00000000000000000 ) ) ;
#6290=PRODUCT_DEFINITION_CONTEXT ( 'detailed design', #8311, 'design' ) ;
#6292=EDGE_CURVE ( 'NONE', #7212, #7915, #7105, .T. ) ;
#6307=DIRECTION ( 'NONE',  ( 1.000000000000000000, 0.000000000000000000, 0.000000000000000000 ) ) ;
#6313=EDGE_CURVE ( 'NONE', #12966, #7287, #543, .T. ) ;
#6352=DIRECTION ( 'NONE',  ( -0.000000000000000000, 0.000000000000000000, -1.000000000000000000 ) ) ;
#6421=CYLINDRICAL_SURFACE ( 'NONE', #8636, 5.000000000000004441 ) ;
#6443=ORIENTED_EDGE ( 'NONE', *, *, #8961, .F. ) ;
#6450=EDGE_LOOP ( 'NONE', ( #8493, #9799 ) ) ;
#6459=CARTESIAN_POINT ( 'NONE',  ( -304.9999999999999432, 45.00000000000001421, 40.00000000000000000 ) ) ;
#6476=CARTESIAN_POINT ( 'NONE',  ( -144.9999999999999432, 55.00000000000001421, 40.00000000000000000 ) ) ;
#6481=CARTESIAN_POINT ( 'NONE',  ( -302.3499999999999659, 45.00000000000001421, 40.00000000000000000 ) ) ;
#6486=VECTOR ( 'NONE', #2577, 1000.000000000000000 ) ;
#6564=AXIS2_PLACEMENT_3D ( 'NONE', #13446, #5124, #8366 ) ;
#6573=ORIENTED_EDGE ( 'NONE', *, *, #1512, .F. ) ;
#6587=EDGE_CURVE ( 'NONE', #7398, #12108, #3799, .T. ) ;
#6588=CARTESIAN_POINT ( 'NONE',  ( -304.9999999999999432, -75.00000000000008527, 354.1421356237308942 ) ) ;
#6598=VERTEX_POINT ( 'NONE', #13730 ) ;
#6605=SHAPE_REPRESENTATION_RELATIONSHIP ( 'NONE' , 'NONE' ,  #9778, #9567 ) ;
#6618=DIRECTION ( 'NONE',  ( -0.000000000000000000, -0.000000000000000000, -1.000000000000000000 ) ) ;
#6637=AXIS2_PLACEMENT_3D ( 'NONE', #7756, #8646, #7617 ) ;
#6648=AXIS2_PLACEMENT_3D ( 'NONE', #1569, #9422, #2609 ) ;
#6667=EDGE_CURVE ( 'NONE', #7915, #5881, #12638, .T. ) ;
#6683=ORIENTED_EDGE ( 'NONE', *, *, #4535, .T. ) ;
#6691=ADVANCED_FACE ( 'NONE', ( #4966, #12715, #2930, #7343, #11779, #353, #3724, #4824 ), #2787, .T. ) ;
#6713=CARTESIAN_POINT ( 'NONE',  ( -145.0000000000000284, -95.00000000000008527, 30.00000000000000000 ) ) ;
#6717=VECTOR ( 'NONE', #5480, 1000.000000000000000 ) ;
#6733=ORIENTED_EDGE ( 'NONE', *, *, #11986, .F. ) ;
#6752=EDGE_LOOP ( 'NONE', ( #1276, #652, #9543, #7396 ) ) ;
#6755=EDGE_CURVE ( 'NONE', #981, #13072, #5462, .T. ) ;
#6762=DIRECTION ( 'NONE',  ( 0.000000000000000000, -0.000000000000000000, 1.000000000000000000 ) ) ;
#6793=VECTOR ( 'NONE', #1725, 1000.000000000000000 ) ;
#6799=CARTESIAN_POINT ( 'NONE',  ( -299.9999999999999432, -95.00000000000008527, 30.00000000000002842 ) ) ;
#6808=ORIENTED_EDGE ( 'NONE', *, *, #9552, .F. ) ;
#6840=ORIENTED_EDGE ( 'NONE', *, *, #8961, .T. ) ;
#6849=FACE_OUTER_BOUND ( 'NONE', #12992, .T. ) ;
#6871=AXIS2_PLACEMENT_3D ( 'NONE', #10766, #11927, #1973 ) ;
#6912=CARTESIAN_POINT ( 'NONE',  ( -299.9999999999999432, -95.00000000000008527, 39.99999999999997868 ) ) ;
#6914=EDGE_CURVE ( 'NONE', #11936, #13138, #1034, .T. ) ;
#6918=CARTESIAN_POINT ( 'NONE',  ( -222.6499999999998920, -85.00000000000009948, 30.00000000000000000 ) ) ;
#6920=AXIS2_PLACEMENT_3D ( 'NONE', #13908, #1718, #3120 ) ;
#6927=AXIS2_PLACEMENT_3D ( 'NONE', #8227, #13749, #4917 ) ;
#6935=AXIS2_PLACEMENT_3D ( 'NONE', #224, #4902, #9104 ) ;
#6937=ADVANCED_FACE ( 'NONE', ( #10093 ), #1160, .F. ) ;
#6943=DIRECTION ( 'NONE',  ( -1.000000000000000000, -1.460819769243627131E-16, 0.000000000000000000 ) ) ;
#6980=ORIENTED_EDGE ( 'NONE', *, *, #5366, .T. ) ;
#7060=DIRECTION ( 'NONE',  ( -1.000000000000000000, 0.000000000000000000, 0.000000000000000000 ) ) ;
#7071=CYLINDRICAL_SURFACE ( 'NONE', #13374, 5.000000000000004441 ) ;
#7086=DIRECTION ( 'NONE',  ( -1.000000000000000000, 0.000000000000000000, 0.000000000000000000 ) ) ;
#7099=EDGE_CURVE ( 'NONE', #8115, #2239, #6167, .T. ) ;
#7105=CIRCLE ( 'NONE', #6648, 5.000000000000004441 ) ;
#7126=AXIS2_PLACEMENT_3D ( 'NONE', #11170, #1214, #250 ) ;
#7129=CARTESIAN_POINT ( 'NONE',  ( -294.9999999999999432, 55.00000000000001421, 40.00000000000000000 ) ) ;
#7212=VERTEX_POINT ( 'NONE', #10748 ) ;
#7219=ORIENTED_EDGE ( 'NONE', *, *, #10381, .F. ) ;
#7231=VECTOR ( 'NONE', #3464, 1000.000000000000000 ) ;
#7237=VECTOR ( 'NONE', #11460, 1000.000000000000000 ) ;
#7271=CARTESIAN_POINT ( 'NONE',  ( -124.9999999999999432, 55.00000000000001421, 40.00000000000000000 ) ) ;
#7273=CARTESIAN_POINT ( 'NONE',  ( -145.0000000000000284, -75.00000000000008527, -14.14213562373090127 ) ) ;
#7283=EDGE_CURVE ( 'NONE', #8115, #663, #4775, .T. ) ;
#7287=VERTEX_POINT ( 'NONE', #7606 ) ;
#7323=FACE_OUTER_BOUND ( 'NONE', #12449, .T. ) ;
#7329=EDGE_CURVE ( 'NONE', #1810, #417, #7777, .T. ) ;
#7341=PLANE ( 'NONE',  #6871 ) ;
#7343=FACE_BOUND ( 'NONE', #477, .T. ) ;
#7352=DIRECTION ( 'NONE',  ( -0.000000000000000000, -0.000000000000000000, -1.000000000000000000 ) ) ;
#7358=DIRECTION ( 'NONE',  ( 1.000000000000000000, 0.000000000000000000, 0.000000000000000000 ) ) ;
#7396=ORIENTED_EDGE ( 'NONE', *, *, #5081, .F. ) ;
#7398=VERTEX_POINT ( 'NONE', #1353 ) ;
#7441=DIRECTION ( 'NONE',  ( 0.000000000000000000, -0.000000000000000000, 1.000000000000000000 ) ) ;
#7448=( GEOMETRIC_REPRESENTATION_CONTEXT ( 3 ) GLOBAL_UNCERTAINTY_ASSIGNED_CONTEXT ( ( #4359 ) ) GLOBAL_UNIT_ASSIGNED_CONTEXT ( ( #7754, #13477, #12055 ) ) REPRESENTATION_CONTEXT ( 'NONE', 'WORKASPACE' ) );
#7460=ORIENTED_EDGE ( 'NONE', *, *, #14290, .T. ) ;
#7465=VECTOR ( 'NONE', #11923, 1000.000000000000000 ) ;
#7483=DIRECTION ( 'NONE',  ( -0.000000000000000000, 0.000000000000000000, -1.000000000000000000 ) ) ;
#7489=CARTESIAN_POINT ( 'NONE',  ( -314.9999999999999432, 55.00000000000001421, 40.00000000000000000 ) ) ;
#7494=DIRECTION ( 'NONE',  ( 1.000000000000000000, 0.000000000000000000, 0.000000000000000000 ) ) ;
#7527=ORIENTED_EDGE ( 'NONE', *, *, #5920, .T. ) ;
#7544=ORIENTED_EDGE ( 'NONE', *, *, #4456, .F. ) ;
#7549=EDGE_CURVE ( 'NONE', #7398, #4493, #8171, .T. ) ;
#7554=DIRECTION ( 'NONE',  ( -0.000000000000000000, -0.000000000000000000, -1.000000000000000000 ) ) ;
#7606=CARTESIAN_POINT ( 'NONE',  ( -294.9999999999999432, -95.00000000000008527, 30.00000000000002842 ) ) ;
#7617=DIRECTION ( 'NONE',  ( 1.000000000000000000, 0.000000000000000000, 0.000000000000000000 ) ) ;
#7648=LINE ( 'NONE', #12083, #3211 ) ;
#7655=CARTESIAN_POINT ( 'NONE',  ( -302.3499999999999659, 45.00000000000001421, 30.00000000000000000 ) ) ;
#7685=CARTESIAN_POINT ( 'NONE',  ( -314.9999999999999432, 55.00000000000001421, 40.00000000000000000 ) ) ;
#7714=VERTEX_POINT ( 'NONE', #5218 ) ;
#7717=DIRECTION ( 'NONE',  ( 0.000000000000000000, -0.000000000000000000, 1.000000000000000000 ) ) ;
#7720=ORIENTED_EDGE ( 'NONE', *, *, #14290, .F. ) ;
#7731=DIRECTION ( 'NONE',  ( 0.000000000000000000, 0.000000000000000000, -1.000000000000000000 ) ) ;
#7754=( LENGTH_UNIT ( ) NAMED_UNIT ( * ) SI_UNIT ( .MILLI., .METRE. ) );
#7756=CARTESIAN_POINT ( 'NONE',  ( -140.0000000000000000, -95.00000000000008527, 30.00000000000000000 ) ) ;
#7758=ORIENTED_EDGE ( 'NONE', *, *, #6587, .F. ) ;
#7763=EDGE_LOOP ( 'NONE', ( #9768, #14181, #12229, #11557 ) ) ;
#7777=CIRCLE ( 'NONE', #8235, 2.649999999999985700 ) ;
#7779=CARTESIAN_POINT ( 'NONE',  ( -144.9999999999999432, 55.00000000000001421, 30.00000000000000000 ) ) ;
#7792=ORIENTED_EDGE ( 'NONE', *, *, #1377, .F. ) ;
#7801=CARTESIAN_POINT ( 'NONE',  ( -314.9999999999999432, -105.0000000000000995, 30.00000000000000000 ) ) ;
#7803=VECTOR ( 'NONE', #3953, 1000.000000000000000 ) ;
#7804=EDGE_CURVE ( 'NONE', #6598, #7398, #3727, .T. ) ;
#7806=STYLED_ITEM('',(#14403),#8473);
#7915=VERTEX_POINT ( 'NONE', #5979 ) ;
#7927=CARTESIAN_POINT ( 'NONE',  ( -124.9999999999999432, -105.0000000000000853, 40.00000000000000000 ) ) ;
#7936=CARTESIAN_POINT ( 'NONE',  ( -124.9999999999999432, 55.00000000000001421, 40.00000000000000000 ) ) ;
#7949=ORIENTED_EDGE ( 'NONE', *, *, #11065, .F. ) ;
#7980=ADVANCED_FACE ( 'NONE', ( #508 ), #8290, .F. ) ;
#7983=FACE_OUTER_BOUND ( 'NONE', #136, .T. ) ;
#8006=VERTEX_POINT ( 'NONE', #12796 ) ;
#8078=ORIENTED_EDGE ( 'NONE', *, *, #9646, .T. ) ;
#8087=DIRECTION ( 'NONE',  ( 1.000000000000000000, 0.000000000000000000, 0.000000000000000000 ) ) ;
#8088=FACE_OUTER_BOUND ( 'NONE', #10231, .T. ) ;
#8115=VERTEX_POINT ( 'NONE', #6481 ) ;
#8121=DIRECTION ( 'NONE',  ( -0.000000000000000000, -0.000000000000000000, -1.000000000000000000 ) ) ;
#8139=CARTESIAN_POINT ( 'NONE',  ( 0.000000000000000000, 0.000000000000000000, 40.00000000000000000 ) ) ;
#8152=CARTESIAN_POINT ( 'NONE',  ( -294.9999999999999432, -65.00000000000011369, 40.00000000000000000 ) ) ;
#8155=CARTESIAN_POINT ( 'NONE',  ( -140.0000000000000000, -75.00000000000008527, -14.14213562373090127 ) ) ;
#8164=FACE_OUTER_BOUND ( 'NONE', #820, .T. ) ;
#8171=LINE ( 'NONE', #11519, #5700 ) ;
#8178=CARTESIAN_POINT ( 'NONE',  ( -137.6499999999999773, 45.00000000000001421, 30.00000000000000000 ) ) ;
#8183=CYLINDRICAL_SURFACE ( 'NONE', #9628, 5.000000000000004441 ) ;
#8204=EDGE_CURVE ( 'NONE', #2540, #4912, #9673, .T. ) ;
#8207=ORIENTED_EDGE ( 'NONE', *, *, #8645, .F. ) ;
#8227=CARTESIAN_POINT ( 'NONE',  ( -314.9999999999999432, 55.00000000000001421, 40.00000000000000000 ) ) ;
#8235=AXIS2_PLACEMENT_3D ( 'NONE', #5509, #248, #103 ) ;
#8269=ORIENTED_EDGE ( 'NONE', *, *, #11039, .F. ) ;
#8288=DIRECTION ( 'NONE',  ( 0.000000000000000000, -0.000000000000000000, 1.000000000000000000 ) ) ;
#8290=CYLINDRICAL_SURFACE ( 'NONE', #1530, 2.649999999999985700 ) ;
#8300=DIRECTION ( 'NONE',  ( 1.000000000000000000, 0.000000000000000000, 0.000000000000000000 ) ) ;
#8311=APPLICATION_CONTEXT ( 'automotive_design' ) ;
#8317=EDGE_CURVE ( 'NONE', #7714, #2336, #8500, .T. ) ;
#8331=CARTESIAN_POINT ( 'NONE',  ( -294.9999999999999432, -105.0000000000000853, 30.00000000000000000 ) ) ;
#8366=DIRECTION ( 'NONE',  ( 1.000000000000000000, 1.460819769243627131E-16, 0.000000000000000000 ) ) ;
#8423=ORIENTED_EDGE ( 'NONE', *, *, #13739, .T. ) ;
#8448=EDGE_CURVE ( 'NONE', #3716, #4493, #4218, .T. ) ;
#8473=MANIFOLD_SOLID_BREP ( 'M5 Clearance Hole2', #3810 ) ;
#8493=ORIENTED_EDGE ( 'NONE', *, *, #6292, .F. ) ;
#8500=CIRCLE ( 'NONE', #2248, 2.649999999999985700 ) ;
#8516=VECTOR ( 'NONE', #5771, 1000.000000000000000 ) ;
#8521=CARTESIAN_POINT ( 'NONE',  ( -299.9999999999999432, -95.00000000000008527, 30.00000000000002842 ) ) ;
#8526=EDGE_LOOP ( 'NONE', ( #11898, #10981, #13665, #10084, #9045, #7544, #11205, #39 ) ) ;
#8571=CARTESIAN_POINT ( 'NONE',  ( -124.9999999999999432, -65.00000000000008527, 40.00000000000000000 ) ) ;
#8574=DIRECTION ( 'NONE',  ( 1.000000000000000000, 0.000000000000000000, 0.000000000000000000 ) ) ;
#8591=EDGE_LOOP ( 'NONE', ( #5532, #2801, #1781, #10552 ) ) ;
#8636=AXIS2_PLACEMENT_3D ( 'NONE', #9761, #10781, #7358 ) ;
#8645=EDGE_CURVE ( 'NONE', #10577, #5028, #2262, .T. ) ;
#8646=DIRECTION ( 'NONE',  ( -0.000000000000000000, 0.000000000000000000, -1.000000000000000000 ) ) ;
#8672=PLANE ( 'NONE',  #9301 ) ;
#8674=CARTESIAN_POINT ( 'NONE',  ( -217.3499999999999375, -85.00000000000009948, 40.00000000000000000 ) ) ;
#8695=CARTESIAN_POINT ( 'NONE',  ( -304.9999999999999432, -75.00000000000008527, 30.00000000000002842 ) ) ;
#8697=AXIS2_PLACEMENT_3D ( 'NONE', #12483, #6618, #11052 ) ;
#8716=DIRECTION ( 'NONE',  ( -0.000000000000000000, 0.000000000000000000, -1.000000000000000000 ) ) ;
#8729=AXIS2_PLACEMENT_3D ( 'NONE', #11138, #5471, #2355 ) ;
#8762=LINE ( 'NONE', #6588, #1122 ) ;
#8846=EDGE_LOOP ( 'NONE', ( #11395, #2137, #10028, #7460 ) ) ;
#8854=VECTOR ( 'NONE', #5758, 1000.000000000000000 ) ;
#8861=CIRCLE ( 'NONE', #13256, 2.649999999999985700 ) ;
#8863=DIRECTION ( 'NONE',  ( 0.000000000000000000, 1.000000000000000000, 0.000000000000000000 ) ) ;
#8891=EDGE_CURVE ( 'NONE', #13194, #12598, #11812, .T. ) ;
#8961=EDGE_CURVE ( 'NONE', #7287, #1982, #1300, .T. ) ;
#8964=DIRECTION ( 'NONE',  ( 1.000000000000000000, -0.000000000000000000, -0.000000000000000000 ) ) ;
#8970=DIRECTION ( 'NONE',  ( 0.000000000000000000, 1.000000000000000000, 0.000000000000000000 ) ) ;
#8996=EDGE_LOOP ( 'NONE', ( #3123, #2779, #3040, #5534 ) ) ;
#9019=ORIENTED_EDGE ( 'NONE', *, *, #7283, .F. ) ;
#9037=EDGE_CURVE ( 'NONE', #663, #8115, #3864, .T. ) ;
#9045=ORIENTED_EDGE ( 'NONE', *, *, #110, .T. ) ;
#9091=DIRECTION ( 'NONE',  ( 1.000000000000000000, -0.000000000000000000, 0.000000000000000000 ) ) ;
#9099=DIRECTION ( 'NONE',  ( 0.000000000000000000, 0.000000000000000000, -1.000000000000000000 ) ) ;
#9104=DIRECTION ( 'NONE',  ( -1.000000000000000000, 0.000000000000000000, 0.000000000000000000 ) ) ;
#9113=DIRECTION ( 'NONE',  ( -0.000000000000000000, 0.000000000000000000, -1.000000000000000000 ) ) ;
#9141=EDGE_LOOP ( 'NONE', ( #10747, #14088 ) ) ;
#9146=ORIENTED_EDGE ( 'NONE', *, *, #13739, .F. ) ;
#9176=CIRCLE ( 'NONE', #5705, 5.000000000000004441 ) ;
#9181=DIRECTION ( 'NONE',  ( 0.000000000000000000, -0.000000000000000000, 1.000000000000000000 ) ) ;
#9227=EDGE_CURVE ( 'NONE', #14079, #4256, #2125, .T. ) ;
#9233=VECTOR ( 'NONE', #7352, 1000.000000000000000 ) ;
#9234=ADVANCED_FACE ( 'NONE', ( #3106, #3963, #4257, #1773, #9476, #1993, #3028, #14033 ), #8672, .F. ) ;
#9239=DIRECTION ( 'NONE',  ( 0.000000000000000000, -0.000000000000000000, 1.000000000000000000 ) ) ;
#9252=DIRECTION ( 'NONE',  ( 0.000000000000000000, 0.000000000000000000, 1.000000000000000000 ) ) ;
#9272=DIRECTION ( 'NONE',  ( -0.000000000000000000, -0.000000000000000000, -1.000000000000000000 ) ) ;
#9284=EDGE_LOOP ( 'NONE', ( #12632, #11576 ) ) ;
#9301=AXIS2_PLACEMENT_3D ( 'NONE', #14106, #7441, #13890 ) ;
#9315=CARTESIAN_POINT ( 'NONE',  ( -124.9999999999999432, -105.0000000000000853, 40.00000000000000000 ) ) ;
#9323=ORIENTED_EDGE ( 'NONE', *, *, #13310, .T. ) ;
#9342=ADVANCED_FACE ( 'NONE', ( #6849 ), #10969, .F. ) ;
#9386=CARTESIAN_POINT ( 'NONE',  ( -219.9999999999999147, -85.00000000000009948, 30.00000000000000000 ) ) ;
#9418=DIRECTION ( 'NONE',  ( 0.000000000000000000, 0.000000000000000000, 1.000000000000000000 ) ) ;
#9422=DIRECTION ( 'NONE',  ( -0.000000000000000000, 0.000000000000000000, -1.000000000000000000 ) ) ;
#9424=AXIS2_PLACEMENT_3D ( 'NONE', #8139, #9239, #13652 ) ;
#9436=VERTEX_POINT ( 'NONE', #11350 ) ;
#9473=DIRECTION ( 'NONE',  ( 1.000000000000000000, 0.000000000000000000, 0.000000000000000000 ) ) ;
#9475=VECTOR ( 'NONE', #998, 1000.000000000000000 ) ;
#9476=FACE_BOUND ( 'NONE', #6450, .T. ) ;
#9508=ORIENTED_EDGE ( 'NONE', *, *, #5925, .T. ) ;
#9536=VECTOR ( 'NONE', #7731, 1000.000000000000000 ) ;
#9543=ORIENTED_EDGE ( 'NONE', *, *, #3339, .T. ) ;
#9552=EDGE_CURVE ( 'NONE', #10577, #1810, #2505, .T. ) ;
#9564=VERTEX_POINT ( 'NONE', #3764 ) ;
#9567=ADVANCED_BREP_SHAPE_REPRESENTATION ( '', ( #8473, #14039 ), #4479 ) ;
#9572=CARTESIAN_POINT ( 'NONE',  ( -294.9999999999999432, -105.0000000000000853, 40.00000000000000000 ) ) ;
#9583=ORIENTED_EDGE ( 'NONE', *, *, #8448, .F. ) ;
#9587=CYLINDRICAL_SURFACE ( 'NONE', #5259, 2.649999999999985700 ) ;
#9601=EDGE_LOOP ( 'NONE', ( #6733, #6443 ) ) ;
#9622=DIRECTION ( 'NONE',  ( -0.000000000000000000, -0.000000000000000000, -1.000000000000000000 ) ) ;
#9628=AXIS2_PLACEMENT_3D ( 'NONE', #11601, #547, #4057 ) ;
#9646=EDGE_CURVE ( 'NONE', #12598, #12063, #14282, .T. ) ;
#9647=CARTESIAN_POINT ( 'NONE',  ( -299.9999999999999432, -95.00000000000008527, 39.99999999999997868 ) ) ;
#9656=CIRCLE ( 'NONE', #6637, 5.000000000000004441 ) ;
#9657=DIRECTION ( 'NONE',  ( -0.000000000000000000, -1.000000000000000000, -0.000000000000000000 ) ) ;
#9667=ORIENTED_EDGE ( 'NONE', *, *, #11704, .T. ) ;
#9673=CIRCLE ( 'NONE', #608, 5.000000000000004441 ) ;
#9708=CARTESIAN_POINT ( 'NONE',  ( -145.0000000000000284, -95.00000000000008527, 40.00000000000000000 ) ) ;
#9717=DIRECTION ( 'NONE',  ( -0.000000000000000000, -0.000000000000000000, -1.000000000000000000 ) ) ;
#9761=CARTESIAN_POINT ( 'NONE',  ( -140.0000000000000000, -95.00000000000008527, -14.14213562373090127 ) ) ;
#9768=ORIENTED_EDGE ( 'NONE', *, *, #8317, .T. ) ;
#9778=SHAPE_REPRESENTATION ( 'aligner', ( #14039 ), #4479 ) ;
#9799=ORIENTED_EDGE ( 'NONE', *, *, #4387, .F. ) ;
#9816=CARTESIAN_POINT ( 'NONE',  ( -124.9999999999999432, -105.0000000000000853, 30.00000000000000000 ) ) ;
#9868=UNCERTAINTY_MEASURE_WITH_UNIT (LENGTH_MEASURE( 1.000000000000000082E-05 ), #5519, 'distance_accuracy_value', 'NONE');
#9892=CIRCLE ( 'NONE', #354, 5.000000000000004441 ) ;
#9904=EDGE_LOOP ( 'NONE', ( #5523, #10852, #2853, #7219 ) ) ;
#9923=CARTESIAN_POINT ( 'NONE',  ( -314.9999999999999432, -105.0000000000000995, 40.00000000000000000 ) ) ;
#9963=CARTESIAN_POINT ( 'NONE',  ( -299.9999999999999432, -75.00000000000008527, 39.99999999999997868 ) ) ;
#9990=CARTESIAN_POINT ( 'NONE',  ( -144.9999999999999432, -65.00000000000008527, 40.00000000000000000 ) ) ;
#10028=ORIENTED_EDGE ( 'NONE', *, *, #5081, .T. ) ;
#10033=ORIENTED_EDGE ( 'NONE', *, *, #9037, .F. ) ;
#10052=EDGE_CURVE ( 'NONE', #12598, #12386, #5843, .T. ) ;
#10083=EDGE_CURVE ( 'NONE', #12108, #12386, #5697, .T. ) ;
#10084=ORIENTED_EDGE ( 'NONE', *, *, #8891, .F. ) ;
#10093=FACE_OUTER_BOUND ( 'NONE', #2613, .T. ) ;
#10112=AXIS2_PLACEMENT_3D ( 'NONE', #1631, #1414, #11439 ) ;
#10117=FACE_OUTER_BOUND ( 'NONE', #14090, .T. ) ;
#10136=( GEOMETRIC_REPRESENTATION_CONTEXT ( 3 ) GLOBAL_UNCERTAINTY_ASSIGNED_CONTEXT ( ( #11855 ) ) GLOBAL_UNIT_ASSIGNED_CONTEXT ( ( #852, #11032, #13124 ) ) REPRESENTATION_CONTEXT ( 'NONE', 'WORKASPACE' ) );
#10158=CARTESIAN_POINT ( 'NONE',  ( -135.0000000000000000, -75.00000000000008527, -14.14213562373090127 ) ) ;
#10179=EDGE_LOOP ( 'NONE', ( #14114, #2265 ) ) ;
#10195=VECTOR ( 'NONE', #499, 1000.000000000000000 ) ;
#10197=CARTESIAN_POINT ( 'NONE',  ( -145.0000000000000284, -95.00000000000008527, -14.14213562373090127 ) ) ;
#10208=ORIENTED_EDGE ( 'NONE', *, *, #5278, .T. ) ;
#10213=ORIENTED_EDGE ( 'NONE', *, *, #11550, .F. ) ;
#10231=EDGE_LOOP ( 'NONE', ( #7949, #2112, #13821, #3019 ) ) ;
#10266=APPLICATION_CONTEXT ( 'automotive_design' ) ;
#10284=ADVANCED_FACE ( 'NONE', ( #10712 ), #741, .F. ) ;
#10288=CARTESIAN_POINT ( 'NONE',  ( -294.9999999999999432, -95.00000000000008527, 354.1421356237308942 ) ) ;
#10294=EDGE_CURVE ( 'NONE', #2887, #1982, #12588, .T. ) ;
#10381=EDGE_CURVE ( 'NONE', #2540, #13072, #10996, .T. ) ;
#10442=DIRECTION ( 'NONE',  ( -0.000000000000000000, -0.000000000000000000, -1.000000000000000000 ) ) ;
#10446=FACE_OUTER_BOUND ( 'NONE', #2909, .T. ) ;
#10462=VERTEX_POINT ( 'NONE', #2064 ) ;
#10495=COLOUR_RGB ( '',0.8941176470588234615, 0.8941176470588234615, 0.8941176470588234615 ) ;
#10508=CARTESIAN_POINT ( 'NONE',  ( 0.000000000000000000, 0.000000000000000000, 0.000000000000000000 ) ) ;
#10543=ORIENTED_EDGE ( 'NONE', *, *, #7804, .F. ) ;
#10552=ORIENTED_EDGE ( 'NONE', *, *, #238, .F. ) ;
#10562=DIRECTION ( 'NONE',  ( 0.000000000000000000, 0.000000000000000000, 1.000000000000000000 ) ) ;
#10572=ADVANCED_FACE ( 'NONE', ( #1987 ), #6421, .F. ) ;
#10577=VERTEX_POINT ( 'NONE', #11937 ) ;
#10586=VECTOR ( 'NONE', #4861, 1000.000000000000000 ) ;
#10712=FACE_OUTER_BOUND ( 'NONE', #7763, .T. ) ;
#10741=CARTESIAN_POINT ( 'NONE',  ( -140.0000000000000000, -75.00000000000008527, 40.00000000000000000 ) ) ;
#10747=ORIENTED_EDGE ( 'NONE', *, *, #12534, .F. ) ;
#10748=CARTESIAN_POINT ( 'NONE',  ( -135.0000000000000000, -75.00000000000008527, 30.00000000000000000 ) ) ;
#10749=DIRECTION ( 'NONE',  ( -0.000000000000000000, -0.000000000000000000, -1.000000000000000000 ) ) ;
#10757=DIRECTION ( 'NONE',  ( 1.000000000000000000, 0.000000000000000000, 0.000000000000000000 ) ) ;
#10760=LINE ( 'NONE', #8571, #11228 ) ;
#10761=ORIENTED_EDGE ( 'NONE', *, *, #10853, .T. ) ;
#10766=CARTESIAN_POINT ( 'NONE',  ( -124.9999999999999432, -105.0000000000000853, 40.00000000000000000 ) ) ;
#10781=DIRECTION ( 'NONE',  ( 0.000000000000000000, -0.000000000000000000, 1.000000000000000000 ) ) ;
#10782=DIRECTION ( 'NONE',  ( 1.000000000000000000, 0.000000000000000000, 0.000000000000000000 ) ) ;
#10783=CARTESIAN_POINT ( 'NONE',  ( -135.0000000000000000, -95.00000000000008527, -14.14213562373090127 ) ) ;
#10784=VECTOR ( 'NONE', #12401, 1000.000000000000000 ) ;
#10831=VECTOR ( 'NONE', #575, 1000.000000000000000 ) ;
#10844=AXIS2_PLACEMENT_3D ( 'NONE', #13156, #11060, #3373 ) ;
#10852=ORIENTED_EDGE ( 'NONE', *, *, #12960, .T. ) ;
#10853=EDGE_CURVE ( 'NONE', #7714, #4256, #11269, .T. ) ;
#10855=EDGE_LOOP ( 'NONE', ( #10033, #9019 ) ) ;
#10858=EDGE_CURVE ( 'NONE', #8006, #11938, #4675, .T. ) ;
#10885=ORIENTED_EDGE ( 'NONE', *, *, #1878, .T. ) ;
#10969=PLANE ( 'NONE',  #6057 ) ;
#10972=PRESENTATION_STYLE_ASSIGNMENT (( #11174 ) ) ;
#10981=ORIENTED_EDGE ( 'NONE', *, *, #10083, .T. ) ;
#10982=CARTESIAN_POINT ( 'NONE',  ( -299.9999999999999432, -75.00000000000008527, 354.1421356237308942 ) ) ;
#10984=CARTESIAN_POINT ( 'NONE',  ( -140.0000000000000000, -95.00000000000008527, 40.00000000000000000 ) ) ;
#10996=LINE ( 'NONE', #10783, #1191 ) ;
#10998=ORIENTED_EDGE ( 'NONE', *, *, #9552, .T. ) ;
#11028=EDGE_CURVE ( 'NONE', #9436, #5881, #219, .T. ) ;
#11032=( NAMED_UNIT ( * ) PLANE_ANGLE_UNIT ( ) SI_UNIT ( $, .RADIAN. ) );
#11039=EDGE_CURVE ( 'NONE', #2887, #12966, #1649, .T. ) ;
#11052=DIRECTION ( 'NONE',  ( -1.000000000000000000, 0.000000000000000000, 0.000000000000000000 ) ) ;
#11060=DIRECTION ( 'NONE',  ( 0.000000000000000000, -0.000000000000000000, 1.000000000000000000 ) ) ;
#11065=EDGE_CURVE ( 'NONE', #3716, #8006, #5370, .T. ) ;
#11087=CARTESIAN_POINT ( 'NONE',  ( -135.0000000000000000, -95.00000000000008527, 40.00000000000000000 ) ) ;
#11092=DIRECTION ( 'NONE',  ( -0.000000000000000000, -0.000000000000000000, -1.000000000000000000 ) ) ;
#11113=VERTEX_POINT ( 'NONE', #8695 ) ;
#11123=CARTESIAN_POINT ( 'NONE',  ( -134.9999999999999716, 45.00000000000001421, 30.00000000000000000 ) ) ;
#11134=EDGE_LOOP ( 'NONE', ( #12835, #7758, #1875, #4965 ) ) ;
#11138=CARTESIAN_POINT ( 'NONE',  ( -299.9999999999999432, -75.00000000000008527, 30.00000000000002842 ) ) ;
#11157=CARTESIAN_POINT ( 'NONE',  ( -124.9999999999999432, 55.00000000000001421, 30.00000000000000000 ) ) ;
#11164=ORIENTED_EDGE ( 'NONE', *, *, #4492, .T. ) ;
#11165=CARTESIAN_POINT ( 'NONE',  ( -124.9999999999999432, -105.0000000000000853, 30.00000000000000000 ) ) ;
#11170=CARTESIAN_POINT ( 'NONE',  ( -219.9999999999999147, -85.00000000000009948, 40.00000000000000000 ) ) ;
#11174=SURFACE_STYLE_USAGE ( .BOTH. , #12261 ) ;
#11196=EDGE_CURVE ( 'NONE', #865, #9564, #13327, .T. ) ;
#11205=ORIENTED_EDGE ( 'NONE', *, *, #3986, .F. ) ;
#11224=DIRECTION ( 'NONE',  ( 1.000000000000000000, 0.000000000000000000, 0.000000000000000000 ) ) ;
#11228=VECTOR ( 'NONE', #2186, 1000.000000000000000 ) ;
#11269=LINE ( 'NONE', #11677, #6793 ) ;
#11272=DIRECTION ( 'NONE',  ( 1.000000000000000000, 0.000000000000000000, 0.000000000000000000 ) ) ;
#11318=EDGE_CURVE ( 'NONE', #11433, #11938, #609, .T. ) ;
#11350=CARTESIAN_POINT ( 'NONE',  ( -135.0000000000000000, -75.00000000000008527, 40.00000000000000000 ) ) ;
#11364=CARTESIAN_POINT ( 'NONE',  ( -304.9999999999999432, 45.00000000000001421, 40.00000000000000000 ) ) ;
#11395=ORIENTED_EDGE ( 'NONE', *, *, #7099, .F. ) ;
#11433=VERTEX_POINT ( 'NONE', #5215 ) ;
#11439=DIRECTION ( 'NONE',  ( -1.000000000000000000, 0.000000000000000000, 0.000000000000000000 ) ) ;
#11440=ORIENTED_EDGE ( 'NONE', *, *, #10858, .F. ) ;
#11460=DIRECTION ( 'NONE',  ( 0.000000000000000000, -0.000000000000000000, 1.000000000000000000 ) ) ;
#11499=CYLINDRICAL_SURFACE ( 'NONE', #971, 5.000000000000004441 ) ;
#11517=VECTOR ( 'NONE', #1087, 1000.000000000000000 ) ;
#11519=CARTESIAN_POINT ( 'NONE',  ( -314.9999999999999432, -105.0000000000000995, 40.00000000000000000 ) ) ;
#11528=AXIS2_PLACEMENT_3D ( 'NONE', #520, #4982, #10562 ) ;
#11531=CYLINDRICAL_SURFACE ( 'NONE', #1978, 2.649999999999985700 ) ;
#11542=CYLINDRICAL_SURFACE ( 'NONE', #5727, 2.649999999999985700 ) ;
#11550=EDGE_CURVE ( 'NONE', #13194, #11433, #13380, .T. ) ;
#11557=ORIENTED_EDGE ( 'NONE', *, *, #10853, .F. ) ;
#11576=ORIENTED_EDGE ( 'NONE', *, *, #238, .T. ) ;
#11601=CARTESIAN_POINT ( 'NONE',  ( -140.0000000000000000, -75.00000000000008527, -14.14213562373090127 ) ) ;
#11604=DIRECTION ( 'NONE',  ( -0.000000000000000000, -1.000000000000000000, -0.000000000000000000 ) ) ;
#11677=CARTESIAN_POINT ( 'NONE',  ( -137.6499999999999773, 45.00000000000001421, 30.00000000000000000 ) ) ;
#11704=EDGE_CURVE ( 'NONE', #11938, #10462, #367, .T. ) ;
#11707=AXIS2_PLACEMENT_3D ( 'NONE', #4295, #8716, #13136 ) ;
#11710=LINE ( 'NONE', #1691, #9233 ) ;
#11742=DIRECTION ( 'NONE',  ( -0.000000000000000000, -1.000000000000000000, -0.000000000000000000 ) ) ;
#11759=DIRECTION ( 'NONE',  ( 1.000000000000000000, 0.000000000000000000, 0.000000000000000000 ) ) ;
#11760=VECTOR ( 'NONE', #9657, 1000.000000000000000 ) ;
#11769=ORIENTED_EDGE ( 'NONE', *, *, #6914, .T. ) ;
#11779=FACE_BOUND ( 'NONE', #9284, .T. ) ;
#11788=ADVANCED_FACE ( 'NONE', ( #4979 ), #11499, .F. ) ;
#11812=LINE ( 'NONE', #92, #12927 ) ;
#11855=UNCERTAINTY_MEASURE_WITH_UNIT (LENGTH_MEASURE( 1.000000000000000082E-05 ), #852, 'distance_accuracy_value', 'NONE');
#11864=ADVANCED_FACE ( 'NONE', ( #12013 ), #12872, .F. ) ;
#11898=ORIENTED_EDGE ( 'NONE', *, *, #6587, .T. ) ;
#11923=DIRECTION ( 'NONE',  ( 0.000000000000000000, 0.000000000000000000, -1.000000000000000000 ) ) ;
#11927=DIRECTION ( 'NONE',  ( -7.304098846218135653E-17, 1.000000000000000000, 0.000000000000000000 ) ) ;
#11936=VERTEX_POINT ( 'NONE', #740 ) ;
#11937=CARTESIAN_POINT ( 'NONE',  ( -222.6499999999998920, -85.00000000000009948, 40.00000000000000000 ) ) ;
#11938=VERTEX_POINT ( 'NONE', #1766 ) ;
#11976=AXIS2_PLACEMENT_3D ( 'NONE', #11364, #9181, #8087 ) ;
#11986=EDGE_CURVE ( 'NONE', #1982, #7287, #2942, .T. ) ;
#11993=DIRECTION ( 'NONE',  ( -1.000000000000000000, 0.000000000000000000, 0.000000000000000000 ) ) ;
#12002=CARTESIAN_POINT ( 'NONE',  ( -135.0000000000000000, -95.00000000000008527, 30.00000000000000000 ) ) ;
#12013=FACE_OUTER_BOUND ( 'NONE', #4763, .T. ) ;
#12018=EDGE_CURVE ( 'NONE', #11113, #13081, #3627, .T. ) ;
#12037=ORIENTED_EDGE ( 'NONE', *, *, #9646, .F. ) ;
#12040=CARTESIAN_POINT ( 'NONE',  ( -304.9999999999999432, -95.00000000000008527, 30.00000000000002842 ) ) ;
#12050=CARTESIAN_POINT ( 'NONE',  ( -314.9999999999999432, -105.0000000000000995, 30.00000000000000000 ) ) ;
#12055=( NAMED_UNIT ( * ) SI_UNIT ( $, .STERADIAN. ) SOLID_ANGLE_UNIT ( ) );
#12057=CARTESIAN_POINT ( 'NONE',  ( -299.9999999999999432, -75.00000000000008527, 39.99999999999997868 ) ) ;
#12058=ORIENTED_EDGE ( 'NONE', *, *, #1878, .F. ) ;
#12063=VERTEX_POINT ( 'NONE', #7779 ) ;
#12083=CARTESIAN_POINT ( 'NONE',  ( -124.9999999999999432, 55.00000000000001421, 40.00000000000000000 ) ) ;
#12108=VERTEX_POINT ( 'NONE', #1247 ) ;
#12128=LINE ( 'NONE', #7489, #7465 ) ;
#12132=ORIENTED_EDGE ( 'NONE', *, *, #12195, .F. ) ;
#12173=DIRECTION ( 'NONE',  ( 0.000000000000000000, 1.000000000000000000, 0.000000000000000000 ) ) ;
#12189=ORIENTED_EDGE ( 'NONE', *, *, #11986, .T. ) ;
#12195=EDGE_CURVE ( 'NONE', #12966, #2887, #9892, .T. ) ;
#12229=ORIENTED_EDGE ( 'NONE', *, *, #9227, .T. ) ;
#12233=CARTESIAN_POINT ( 'NONE',  ( -294.9999999999999432, -95.00000000000008527, 39.99999999999997868 ) ) ;
#12261=SURFACE_SIDE_STYLE ('',( #109 ) ) ;
#12360=EDGE_LOOP ( 'NONE', ( #10213, #13495, #8078, #9146 ) ) ;
#12366=DIRECTION ( 'NONE',  ( -1.000000000000000000, 0.000000000000000000, 0.000000000000000000 ) ) ;
#12386=VERTEX_POINT ( 'NONE', #7271 ) ;
#12401=DIRECTION ( 'NONE',  ( -0.000000000000000000, -0.000000000000000000, -1.000000000000000000 ) ) ;
#12430=AXIS2_PLACEMENT_3D ( 'NONE', #3021, #6205, #13883 ) ;
#12444=CARTESIAN_POINT ( 'NONE',  ( -140.0000000000000000, -95.00000000000008527, -14.14213562373090127 ) ) ;
#12449=EDGE_LOOP ( 'NONE', ( #5528, #606, #10998, #777 ) ) ;
#12453=ADVANCED_FACE ( 'NONE', ( #2927 ), #7341, .F. ) ;
#12473=ORIENTED_EDGE ( 'NONE', *, *, #8204, .F. ) ;
#12483=CARTESIAN_POINT ( 'NONE',  ( -299.9999999999999432, -95.00000000000008527, 354.1421356237308942 ) ) ;
#12528=ADVANCED_FACE ( 'NONE', ( #4586 ), #13144, .F. ) ;
#12534=EDGE_CURVE ( 'NONE', #4256, #14079, #3639, .T. ) ;
#12537=EDGE_LOOP ( 'NONE', ( #5125, #13606 ) ) ;
#12571=STYLED_ITEM ( 'NONE', ( #10972 ), #9567 ) ;
#12588=LINE ( 'NONE', #13744, #4695 ) ;
#12598=VERTEX_POINT ( 'NONE', #6476 ) ;
#12617=CIRCLE ( 'NONE', #11707, 5.000000000000004441 ) ;
#12618=AXIS2_PLACEMENT_3D ( 'NONE', #1090, #2271, #5609 ) ;
#12622=CARTESIAN_POINT ( 'NONE',  ( -302.3499999999999659, 45.00000000000001421, 30.00000000000000000 ) ) ;
#12632=ORIENTED_EDGE ( 'NONE', *, *, #11028, .T. ) ;
#12638=LINE ( 'NONE', #7273, #13820 ) ;
#12715=FACE_BOUND ( 'NONE', #10855, .T. ) ;
#12789=VECTOR ( 'NONE', #6307, 1000.000000000000000 ) ;
#12796=CARTESIAN_POINT ( 'NONE',  ( -294.9999999999999432, 55.00000000000001421, 30.00000000000000000 ) ) ;
#12835=ORIENTED_EDGE ( 'NONE', *, *, #251, .F. ) ;
#12872=PLANE ( 'NONE',  #12430 ) ;
#12927=VECTOR ( 'NONE', #8970, 1000.000000000000000 ) ;
#12937=DIRECTION ( 'NONE',  ( -0.000000000000000000, -0.000000000000000000, -1.000000000000000000 ) ) ;
#12960=EDGE_CURVE ( 'NONE', #4912, #981, #4620, .T. ) ;
#12966=VERTEX_POINT ( 'NONE', #12233 ) ;
#12992=EDGE_LOOP ( 'NONE', ( #14124, #2468, #2415, #422 ) ) ;
#13072=VERTEX_POINT ( 'NONE', #11087 ) ;
#13081=VERTEX_POINT ( 'NONE', #5563 ) ;
#13087=AXIS2_PLACEMENT_3D ( 'NONE', #1723, #5087, #5158 ) ;
#13117=ADVANCED_FACE ( 'NONE', ( #5061 ), #7071, .F. ) ;
#13124=( NAMED_UNIT ( * ) SI_UNIT ( $, .STERADIAN. ) SOLID_ANGLE_UNIT ( ) );
#13128=CARTESIAN_POINT ( 'NONE',  ( -144.9999999999999432, 55.00000000000001421, 40.00000000000000000 ) ) ;
#13130=ADVANCED_FACE ( 'NONE', ( #13886 ), #592, .T. ) ;
#13136=DIRECTION ( 'NONE',  ( 1.000000000000000000, 0.000000000000000000, 0.000000000000000000 ) ) ;
#13138=VERTEX_POINT ( 'NONE', #1406 ) ;
#13144=CYLINDRICAL_SURFACE ( 'NONE', #14286, 5.000000000000004441 ) ;
#13156=CARTESIAN_POINT ( 'NONE',  ( -134.9999999999999716, 45.00000000000001421, 40.00000000000000000 ) ) ;
#13190=DIRECTION ( 'NONE',  ( 1.000000000000000000, 0.000000000000000000, 0.000000000000000000 ) ) ;
#13194=VERTEX_POINT ( 'NONE', #2949 ) ;
#13195=CIRCLE ( 'NONE', #6935, 2.649999999999985700 ) ;
#13215=LINE ( 'NONE', #9816, #2833 ) ;
#13220=AXIS2_PLACEMENT_3D ( 'NONE', #3321, #9717, #2211 ) ;
#13256=AXIS2_PLACEMENT_3D ( 'NONE', #6256, #14084, #8574 ) ;
#13260=VECTOR ( 'NONE', #8964, 1000.000000000000000 ) ;
#13276=LINE ( 'NONE', #7685, #9475 ) ;
#13310=EDGE_CURVE ( 'NONE', #12386, #9564, #7648, .T. ) ;
#13320=LINE ( 'NONE', #11157, #3246 ) ;
#13327=LINE ( 'NONE', #11165, #4188 ) ;
#13360=EDGE_LOOP ( 'NONE', ( #9583, #13742, #403, #13756, #8423, #11164, #13557, #6573 ) ) ;
#13374=AXIS2_PLACEMENT_3D ( 'NONE', #8155, #6062, #9473 ) ;
#13380=LINE ( 'NONE', #9990, #9536 ) ;
#13381=CARTESIAN_POINT ( 'NONE',  ( -124.9999999999999432, -105.0000000000000853, 40.00000000000000000 ) ) ;
#13387=DIRECTION ( 'NONE',  ( 1.000000000000000000, -0.000000000000000000, -0.000000000000000000 ) ) ;
#13446=CARTESIAN_POINT ( 'NONE',  ( -124.9999999999999432, -65.00000000000008527, 40.00000000000000000 ) ) ;
#13448=ORIENTED_EDGE ( 'NONE', *, *, #1299, .F. ) ;
#13477=( NAMED_UNIT ( * ) PLANE_ANGLE_UNIT ( ) SI_UNIT ( $, .RADIAN. ) );
#13488=LINE ( 'NONE', #3560, #10784 ) ;
#13495=ORIENTED_EDGE ( 'NONE', *, *, #8891, .T. ) ;
#13499=CARTESIAN_POINT ( 'NONE',  ( -134.9999999999999716, 45.00000000000001421, 40.00000000000000000 ) ) ;
#13557=ORIENTED_EDGE ( 'NONE', *, *, #11196, .F. ) ;
#13606=ORIENTED_EDGE ( 'NONE', *, *, #5202, .F. ) ;
#13630=ORIENTED_EDGE ( 'NONE', *, *, #12018, .F. ) ;
#13652=DIRECTION ( 'NONE',  ( 1.000000000000000000, 0.000000000000000000, -0.000000000000000000 ) ) ;
#13665=ORIENTED_EDGE ( 'NONE', *, *, #10052, .F. ) ;
#13683=CARTESIAN_POINT ( 'NONE',  ( -124.9999999999999432, -105.0000000000000853, 30.00000000000000000 ) ) ;
#13718=ORIENTED_EDGE ( 'NONE', *, *, #11039, .T. ) ;
#13730=CARTESIAN_POINT ( 'NONE',  ( -314.9999999999999432, 55.00000000000001421, 40.00000000000000000 ) ) ;
#13739=EDGE_CURVE ( 'NONE', #11433, #12063, #4451, .T. ) ;
#13742=ORIENTED_EDGE ( 'NONE', *, *, #11065, .T. ) ;
#13744=CARTESIAN_POINT ( 'NONE',  ( -304.9999999999999432, -95.00000000000008527, 354.1421356237308942 ) ) ;
#13749=DIRECTION ( 'NONE',  ( -0.000000000000000000, 1.000000000000000000, 0.000000000000000000 ) ) ;
#13756=ORIENTED_EDGE ( 'NONE', *, *, #11318, .F. ) ;
#13808=DIRECTION ( 'NONE',  ( 0.000000000000000000, -0.000000000000000000, 1.000000000000000000 ) ) ;
#13820=VECTOR ( 'NONE', #8288, 1000.000000000000000 ) ;
#13821=ORIENTED_EDGE ( 'NONE', *, *, #3986, .T. ) ;
#13855=EDGE_LOOP ( 'NONE', ( #2679, #7527, #4459, #2401 ) ) ;
#13862=ORIENTED_EDGE ( 'NONE', *, *, #6755, .T. ) ;
#13880=ADVANCED_FACE ( 'NONE', ( #332 ), #11542, .F. ) ;
#13883=DIRECTION ( 'NONE',  ( 0.000000000000000000, 0.000000000000000000, -1.000000000000000000 ) ) ;
#13886=FACE_OUTER_BOUND ( 'NONE', #12360, .T. ) ;
#13890=DIRECTION ( 'NONE',  ( 1.000000000000000000, 0.000000000000000000, -0.000000000000000000 ) ) ;
#13908=CARTESIAN_POINT ( 'NONE',  ( -140.0000000000000000, -75.00000000000008527, 30.00000000000000000 ) ) ;
#13972=VERTEX_POINT ( 'NONE', #5740 ) ;
#14000=ORIENTED_EDGE ( 'NONE', *, *, #5925, .F. ) ;
#14022=AXIS2_PLACEMENT_3D ( 'NONE', #10984, #1975, #7494 ) ;
#14026=CARTESIAN_POINT ( 'NONE',  ( -134.9999999999999716, 45.00000000000001421, 30.00000000000000000 ) ) ;
#14033=FACE_OUTER_BOUND ( 'NONE', #13360, .T. ) ;
#14039=AXIS2_PLACEMENT_3D ( 'NONE', #10508, #9418, #5077 ) ;
#14079=VERTEX_POINT ( 'NONE', #3062 ) ;
#14084=DIRECTION ( 'NONE',  ( 0.000000000000000000, -0.000000000000000000, 1.000000000000000000 ) ) ;
#14088=ORIENTED_EDGE ( 'NONE', *, *, #9227, .F. ) ;
#14090=EDGE_LOOP ( 'NONE', ( #420, #5992, #5075, #9667 ) ) ;
#14106=CARTESIAN_POINT ( 'NONE',  ( 0.000000000000000000, 0.000000000000000000, 30.00000000000000000 ) ) ;
#14110=ADVANCED_FACE ( 'NONE', ( #7323 ), #9587, .F. ) ;
#14114=ORIENTED_EDGE ( 'NONE', *, *, #8317, .F. ) ;
#14124=ORIENTED_EDGE ( 'NONE', *, *, #11196, .T. ) ;
#14165=VECTOR ( 'NONE', #4290, 1000.000000000000000 ) ;
#14181=ORIENTED_EDGE ( 'NONE', *, *, #5068, .T. ) ;
#14205=EDGE_LOOP ( 'NONE', ( #7720, #4124 ) ) ;
#14222=EDGE_LOOP ( 'NONE', ( #14000, #10208, #10885, #5678 ) ) ;
#14250=AXIS2_PLACEMENT_3D ( 'NONE', #9963, #3369, #5667 ) ;
#14262=AXIS2_PLACEMENT_3D ( 'NONE', #312, #1354, #7086 ) ;
#14282=LINE ( 'NONE', #13128, #14165 ) ;
#14286=AXIS2_PLACEMENT_3D ( 'NONE', #10982, #7554, #4379 ) ;
#14290=EDGE_CURVE ( 'NONE', #5230, #2239, #341, .T. ) ;
#14397=COLOUR_RGB('Sky Blue',0.24,0.69,0.87);
#14398=FILL_AREA_STYLE_COLOUR('',#14397);
#14399=FILL_AREA_STYLE('',(#14398));
#14400=SURFACE_STYLE_FILL_AREA(#14399);
#14401=SURFACE_SIDE_STYLE('',(#14400));
#14402=SURFACE_STYLE_USAGE(.BOTH.,#14401);
#14403=PRESENTATION_STYLE_ASSIGNMENT((#14402));
ENDSEC;
END-ISO-10303-21;
